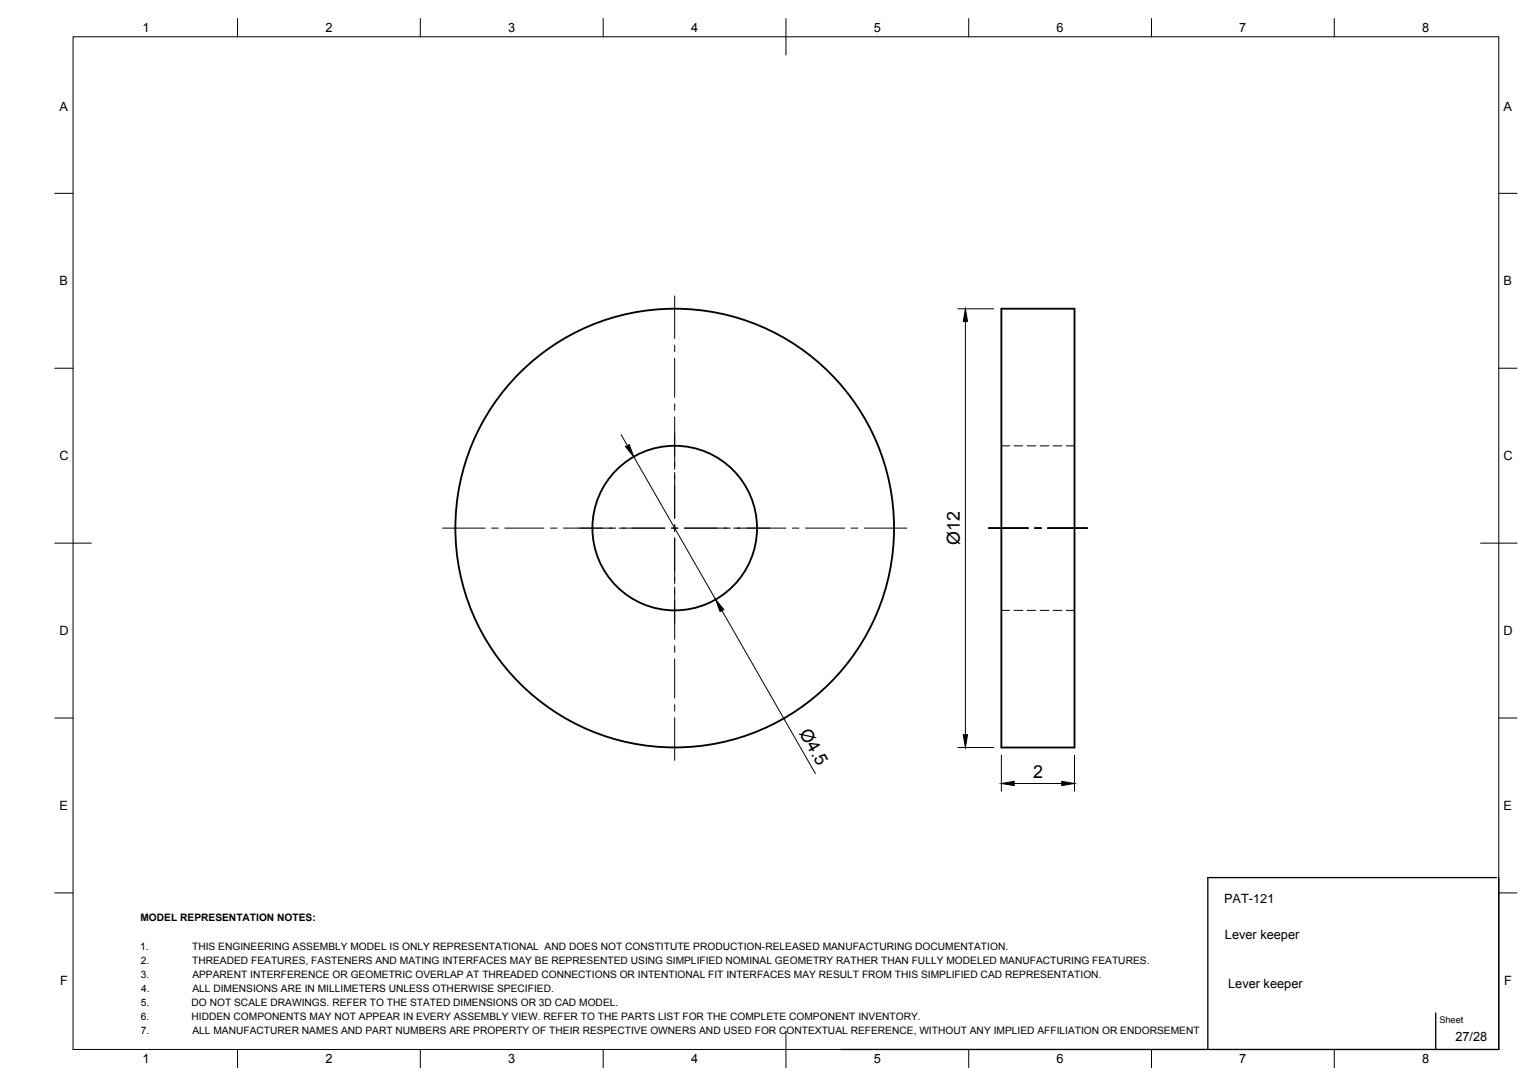
ISO-10303-21;
HEADER;
/* Generated by software containing ST-Developer
 * from STEP Tools, Inc. (www.steptools.com) 
 */

FILE_DESCRIPTION(
/* description */ ('Wall-mounted air drop station'),
/* implementation_level */ '2;1');

FILE_NAME(
/* name */ 'Lever keeper.step',
/* time_stamp */ '2026-10-28T22:16:19-07:00',
/* author */ (''),
/* organization */ (''),
/* preprocessor_version */ 'ST-DEVELOPER v20.2',
/* originating_system */ 'Autodesk Translation Framework v15.17.0.0',
/* authorisation */ '');

FILE_SCHEMA (('AUTOMOTIVE_DESIGN { 1 0 10303 214 3 1 1 }'));
ENDSEC;

DATA;
#10=MECHANICAL_DESIGN_GEOMETRIC_PRESENTATION_REPRESENTATION('',(#370),#10517);
#312=SHAPE_REPRESENTATION_RELATIONSHIP('SRR','None',#10670,#341);
#341=ADVANCED_BREP_SHAPE_REPRESENTATION('',(#397),#10514);
#370=STYLED_ITEM('',(#10867),#397);
#397=MANIFOLD_SOLID_BREP('Body1',#5911);
#523=FACE_BOUND('',#1566,.T.);
#524=FACE_BOUND('',#1568,.T.);
#736=PLANE('',#6883);
#737=PLANE('',#6884);
#1084=FACE_OUTER_BOUND('',#1563,.T.);
#1085=FACE_OUTER_BOUND('',#1564,.T.);
#1086=FACE_OUTER_BOUND('',#1565,.T.);
#1087=FACE_OUTER_BOUND('',#1567,.T.);
#1563=EDGE_LOOP('',(#5335,#5336,#5337,#5338));
#1564=EDGE_LOOP('',(#5339,#5340,#5341,#5342));
#1565=EDGE_LOOP('',(#5343));
#1566=EDGE_LOOP('',(#5344));
#1567=EDGE_LOOP('',(#5345));
#1568=EDGE_LOOP('',(#5346));
#2019=LINE('',#10341,#2483);
#2020=LINE('',#10347,#2484);
#2483=VECTOR('',#8639,0.225);
#2484=VECTOR('',#8646,0.6);
#2754=CIRCLE('',#6878,0.225);
#2755=CIRCLE('',#6879,0.225);
#2756=CIRCLE('',#6881,0.6);
#2757=CIRCLE('',#6882,0.6);
#3213=VERTEX_POINT('',#10338);
#3214=VERTEX_POINT('',#10340);
#3215=VERTEX_POINT('',#10344);
#3216=VERTEX_POINT('',#10346);
#3925=EDGE_CURVE('',#3213,#3213,#2754,.T.);
#3926=EDGE_CURVE('',#3213,#3214,#2019,.T.);
#3927=EDGE_CURVE('',#3214,#3214,#2755,.T.);
#3928=EDGE_CURVE('',#3215,#3215,#2756,.T.);
#3929=EDGE_CURVE('',#3215,#3216,#2020,.T.);
#3930=EDGE_CURVE('',#3216,#3216,#2757,.T.);
#5335=ORIENTED_EDGE('',*,*,#3925,.F.);
#5336=ORIENTED_EDGE('',*,*,#3926,.T.);
#5337=ORIENTED_EDGE('',*,*,#3927,.T.);
#5338=ORIENTED_EDGE('',*,*,#3926,.F.);
#5339=ORIENTED_EDGE('',*,*,#3928,.F.);
#5340=ORIENTED_EDGE('',*,*,#3929,.T.);
#5341=ORIENTED_EDGE('',*,*,#3930,.T.);
#5342=ORIENTED_EDGE('',*,*,#3929,.F.);
#5343=ORIENTED_EDGE('',*,*,#3928,.T.);
#5344=ORIENTED_EDGE('',*,*,#3925,.T.);
#5345=ORIENTED_EDGE('',*,*,#3930,.F.);
#5346=ORIENTED_EDGE('',*,*,#3927,.F.);
#5524=CYLINDRICAL_SURFACE('',#6877,0.225);
#5525=CYLINDRICAL_SURFACE('',#6880,0.6);
#5857=ADVANCED_FACE('',(#1084),#5524,.F.);
#5858=ADVANCED_FACE('',(#1085),#5525,.T.);
#5859=ADVANCED_FACE('',(#1086,#523),#736,.T.);
#5860=ADVANCED_FACE('',(#1087,#524),#737,.F.);
#5911=CLOSED_SHELL('',(#5857,#5858,#5859,#5860));
#6876=AXIS2_PLACEMENT_3D('',#10336,#8633,#8634);
#6877=AXIS2_PLACEMENT_3D('',#10337,#8635,#8636);
#6878=AXIS2_PLACEMENT_3D('',#10339,#8637,#8638);
#6879=AXIS2_PLACEMENT_3D('',#10342,#8640,#8641);
#6880=AXIS2_PLACEMENT_3D('',#10343,#8642,#8643);
#6881=AXIS2_PLACEMENT_3D('',#10345,#8644,#8645);
#6882=AXIS2_PLACEMENT_3D('',#10348,#8647,#8648);
#6883=AXIS2_PLACEMENT_3D('',#10349,#8649,#8650);
#6884=AXIS2_PLACEMENT_3D('',#10350,#8651,#8652);
#8633=DIRECTION('axis',(0.,0.,1.));
#8634=DIRECTION('refdir',(1.,0.,0.));
#8635=DIRECTION('center_axis',(0.,0.,1.));
#8636=DIRECTION('ref_axis',(1.,0.,0.));
#8637=DIRECTION('center_axis',(0.,0.,-1.));
#8638=DIRECTION('ref_axis',(1.,0.,0.));
#8639=DIRECTION('',(0.,0.,-1.));
#8640=DIRECTION('center_axis',(0.,0.,-1.));
#8641=DIRECTION('ref_axis',(1.,0.,0.));
#8642=DIRECTION('center_axis',(0.,0.,1.));
#8643=DIRECTION('ref_axis',(1.,0.,0.));
#8644=DIRECTION('center_axis',(0.,0.,1.));
#8645=DIRECTION('ref_axis',(1.,0.,0.));
#8646=DIRECTION('',(0.,0.,-1.));
#8647=DIRECTION('center_axis',(0.,0.,1.));
#8648=DIRECTION('ref_axis',(1.,0.,0.));
#8649=DIRECTION('center_axis',(0.,0.,1.));
#8650=DIRECTION('ref_axis',(1.,0.,0.));
#8651=DIRECTION('center_axis',(0.,0.,1.));
#8652=DIRECTION('ref_axis',(1.,0.,0.));
#10336=CARTESIAN_POINT('',(0.,0.,0.));
#10337=CARTESIAN_POINT('Origin',(0.,0.,9.4));
#10338=CARTESIAN_POINT('',(-0.225,-2.75545529808154E-17,9.6));
#10339=CARTESIAN_POINT('Origin',(0.,0.,9.6));
#10340=CARTESIAN_POINT('',(-0.225,-2.75545529808154E-17,9.4));
#10341=CARTESIAN_POINT('',(-0.225,-2.75545529808154E-17,9.4));
#10342=CARTESIAN_POINT('Origin',(0.,0.,9.4));
#10343=CARTESIAN_POINT('Origin',(0.,0.,9.4));
#10344=CARTESIAN_POINT('',(-0.6,-7.34788079488412E-17,9.6));
#10345=CARTESIAN_POINT('Origin',(0.,0.,9.6));
#10346=CARTESIAN_POINT('',(-0.6,-7.34788079488412E-17,9.4));
#10347=CARTESIAN_POINT('',(-0.6,-7.34788079488412E-17,9.4));
#10348=CARTESIAN_POINT('Origin',(0.,0.,9.4));
#10349=CARTESIAN_POINT('Origin',(0.,0.,9.6));
#10350=CARTESIAN_POINT('Origin',(0.,0.,9.4));
#10481=UNCERTAINTY_MEASURE_WITH_UNIT(LENGTH_MEASURE(0.001),#10518,
'DISTANCE_ACCURACY_VALUE',
'Maximum model space distance between geometric entities at asserted c
onnectivities');
#10484=UNCERTAINTY_MEASURE_WITH_UNIT(LENGTH_MEASURE(0.001),#10518,
'DISTANCE_ACCURACY_VALUE',
'Maximum model space distance between geometric entities at asserted c
onnectivities');
#10514=(
GEOMETRIC_REPRESENTATION_CONTEXT(3)
GLOBAL_UNCERTAINTY_ASSIGNED_CONTEXT((#10481))
GLOBAL_UNIT_ASSIGNED_CONTEXT((#10518,#10520,#10521))
REPRESENTATION_CONTEXT('','3D')
);
#10517=(
GEOMETRIC_REPRESENTATION_CONTEXT(3)
GLOBAL_UNCERTAINTY_ASSIGNED_CONTEXT((#10484))
GLOBAL_UNIT_ASSIGNED_CONTEXT((#10518,#10520,#10521))
REPRESENTATION_CONTEXT('','3D')
);
#10518=(
LENGTH_UNIT()
NAMED_UNIT(*)
SI_UNIT(.CENTI.,.METRE.)
);
#10520=(
NAMED_UNIT(*)
PLANE_ANGLE_UNIT()
SI_UNIT($,.RADIAN.)
);
#10521=(
NAMED_UNIT(*)
SI_UNIT($,.STERADIAN.)
SOLID_ANGLE_UNIT()
);
#10551=SHAPE_DEFINITION_REPRESENTATION(#10630,#10670);
#10630=PRODUCT_DEFINITION_SHAPE('',$,#10703);
#10670=SHAPE_REPRESENTATION('',(#6876),#10514);
#10673=PRODUCT_DEFINITION_CONTEXT('part definition',#10771,'design');
#10703=PRODUCT_DEFINITION('Lever keeper','Lever keeper',#10735,#10673);
#10735=PRODUCT_DEFINITION_FORMATION('',$,#10802);
#10771=APPLICATION_CONTEXT(
'Core Data for Automotive Mechanical Design Process');
#10772=PRODUCT_CONTEXT('part definition',#10771,'mechanical');
#10802=PRODUCT('Lever keeper','Lever keeper','Lever keeper',(#10772));
#10861=COLOUR_RGB('Sky Blue',0.24,0.69,0.87);
#10862=FILL_AREA_STYLE_COLOUR('',#10861);
#10863=FILL_AREA_STYLE('',(#10862));
#10864=SURFACE_STYLE_FILL_AREA(#10863);
#10865=SURFACE_SIDE_STYLE('',(#10864));
#10866=SURFACE_STYLE_USAGE(.BOTH.,#10865);
#10867=PRESENTATION_STYLE_ASSIGNMENT((#10866));
ENDSEC;
END-ISO-10303-21;
